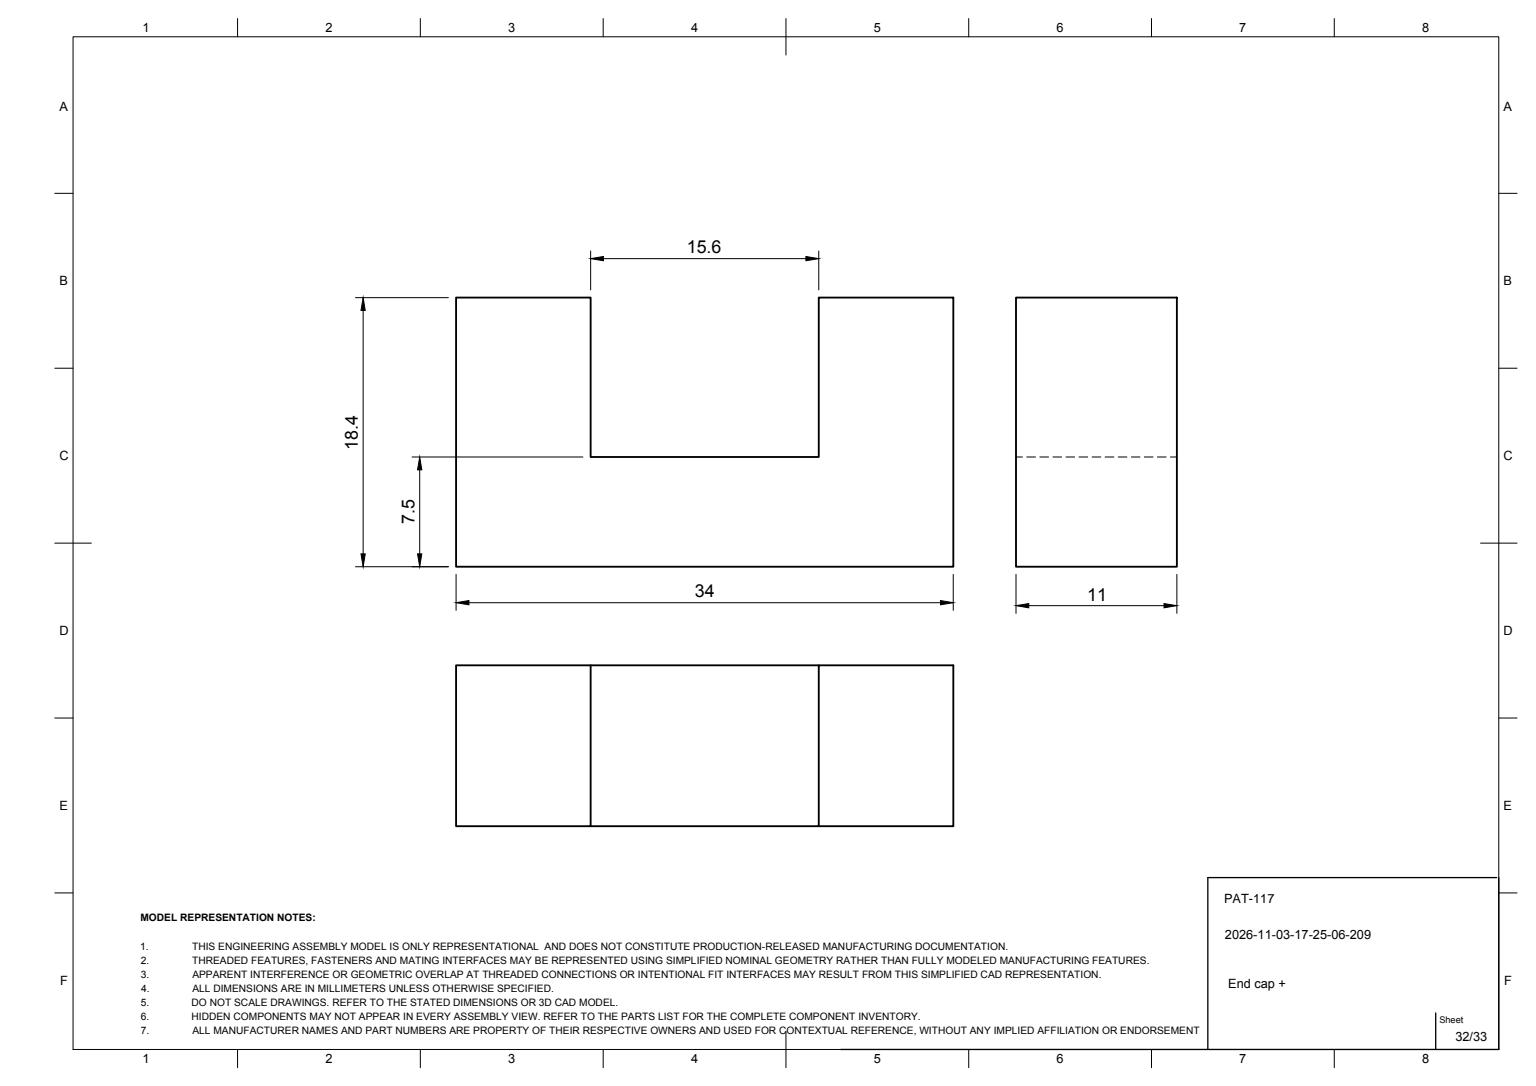
ISO-10303-21;
HEADER;
/* Generated by software containing ST-Developer
 * from STEP Tools, Inc. (www.steptools.com) 
 */

FILE_DESCRIPTION(
/* description */ ('Counterbalanced vertical column'),
/* implementation_level */ '2;1');

FILE_NAME(
/* name */ 'End cap +.step',
/* time_stamp */ '2026-10-29T16:47:22-07:00',
/* author */ (''),
/* organization */ (''),
/* preprocessor_version */ 'ST-DEVELOPER v20.2',
/* originating_system */ 'Autodesk Translation Framework v15.17.0.0',
/* authorisation */ '');

FILE_SCHEMA (('AUTOMOTIVE_DESIGN { 1 0 10303 214 3 1 1 }'));
ENDSEC;

DATA;
#10=MECHANICAL_DESIGN_GEOMETRIC_PRESENTATION_REPRESENTATION('',(#381),#15040);
#311=SHAPE_REPRESENTATION_RELATIONSHIP('SRR','None',#15217,#346);
#346=ADVANCED_BREP_SHAPE_REPRESENTATION('',(#414),#15036);
#381=STYLED_ITEM('',(#15450),#414);
#414=MANIFOLD_SOLID_BREP('Body1',#7106);
#784=PLANE('',#8091);
#785=PLANE('',#8092);
#786=PLANE('',#8093);
#787=PLANE('',#8094);
#788=PLANE('',#8095);
#789=PLANE('',#8096);
#790=PLANE('',#8097);
#791=PLANE('',#8098);
#792=PLANE('',#8099);
#793=PLANE('',#8100);
#1178=FACE_OUTER_BOUND('',#1696,.T.);
#1179=FACE_OUTER_BOUND('',#1697,.T.);
#1180=FACE_OUTER_BOUND('',#1698,.T.);
#1181=FACE_OUTER_BOUND('',#1699,.T.);
#1182=FACE_OUTER_BOUND('',#1700,.T.);
#1183=FACE_OUTER_BOUND('',#1701,.T.);
#1184=FACE_OUTER_BOUND('',#1702,.T.);
#1185=FACE_OUTER_BOUND('',#1703,.T.);
#1186=FACE_OUTER_BOUND('',#1704,.T.);
#1187=FACE_OUTER_BOUND('',#1705,.T.);
#1696=EDGE_LOOP('',(#6354,#6355,#6356,#6357));
#1697=EDGE_LOOP('',(#6358,#6359,#6360,#6361));
#1698=EDGE_LOOP('',(#6362,#6363,#6364,#6365));
#1699=EDGE_LOOP('',(#6366,#6367,#6368,#6369));
#1700=EDGE_LOOP('',(#6370,#6371,#6372,#6373));
#1701=EDGE_LOOP('',(#6374,#6375,#6376,#6377));
#1702=EDGE_LOOP('',(#6378,#6379,#6380,#6381));
#1703=EDGE_LOOP('',(#6382,#6383,#6384,#6385));
#1704=EDGE_LOOP('',(#6386,#6387,#6388,#6389,#6390,#6391,#6392,#6393));
#1705=EDGE_LOOP('',(#6394,#6395,#6396,#6397,#6398,#6399,#6400,#6401));
#2327=LINE('',#14668,#2998);
#2328=LINE('',#14670,#2999);
#2329=LINE('',#14672,#3000);
#2330=LINE('',#14673,#3001);
#2331=LINE('',#14676,#3002);
#2332=LINE('',#14678,#3003);
#2333=LINE('',#14679,#3004);
#2334=LINE('',#14682,#3005);
#2335=LINE('',#14684,#3006);
#2336=LINE('',#14685,#3007);
#2337=LINE('',#14688,#3008);
#2338=LINE('',#14690,#3009);
#2339=LINE('',#14691,#3010);
#2340=LINE('',#14694,#3011);
#2341=LINE('',#14696,#3012);
#2342=LINE('',#14697,#3013);
#2343=LINE('',#14700,#3014);
#2344=LINE('',#14702,#3015);
#2345=LINE('',#14703,#3016);
#2346=LINE('',#14706,#3017);
#2347=LINE('',#14708,#3018);
#2348=LINE('',#14709,#3019);
#2349=LINE('',#14711,#3020);
#2350=LINE('',#14712,#3021);
#2998=VECTOR('',#9985,1.);
#2999=VECTOR('',#9986,1.);
#3000=VECTOR('',#9987,1.);
#3001=VECTOR('',#9988,1.);
#3002=VECTOR('',#9991,1.);
#3003=VECTOR('',#9992,1.);
#3004=VECTOR('',#9993,1.);
#3005=VECTOR('',#9996,1.);
#3006=VECTOR('',#9997,1.);
#3007=VECTOR('',#9998,1.);
#3008=VECTOR('',#10001,1.);
#3009=VECTOR('',#10002,1.);
#3010=VECTOR('',#10003,1.);
#3011=VECTOR('',#10006,1.);
#3012=VECTOR('',#10007,1.);
#3013=VECTOR('',#10008,1.);
#3014=VECTOR('',#10011,1.);
#3015=VECTOR('',#10012,1.);
#3016=VECTOR('',#10013,1.);
#3017=VECTOR('',#10016,1.);
#3018=VECTOR('',#10017,1.);
#3019=VECTOR('',#10018,1.);
#3020=VECTOR('',#10021,1.);
#3021=VECTOR('',#10022,1.);
#3824=VERTEX_POINT('',#14666);
#3825=VERTEX_POINT('',#14667);
#3826=VERTEX_POINT('',#14669);
#3827=VERTEX_POINT('',#14671);
#3828=VERTEX_POINT('',#14675);
#3829=VERTEX_POINT('',#14677);
#3830=VERTEX_POINT('',#14681);
#3831=VERTEX_POINT('',#14683);
#3832=VERTEX_POINT('',#14687);
#3833=VERTEX_POINT('',#14689);
#3834=VERTEX_POINT('',#14693);
#3835=VERTEX_POINT('',#14695);
#3836=VERTEX_POINT('',#14699);
#3837=VERTEX_POINT('',#14701);
#3838=VERTEX_POINT('',#14705);
#3839=VERTEX_POINT('',#14707);
#4678=EDGE_CURVE('',#3824,#3825,#2327,.T.);
#4679=EDGE_CURVE('',#3825,#3826,#2328,.T.);
#4680=EDGE_CURVE('',#3827,#3826,#2329,.T.);
#4681=EDGE_CURVE('',#3824,#3827,#2330,.T.);
#4682=EDGE_CURVE('',#3828,#3824,#2331,.T.);
#4683=EDGE_CURVE('',#3829,#3827,#2332,.T.);
#4684=EDGE_CURVE('',#3828,#3829,#2333,.T.);
#4685=EDGE_CURVE('',#3830,#3828,#2334,.T.);
#4686=EDGE_CURVE('',#3831,#3829,#2335,.T.);
#4687=EDGE_CURVE('',#3830,#3831,#2336,.T.);
#4688=EDGE_CURVE('',#3832,#3830,#2337,.T.);
#4689=EDGE_CURVE('',#3833,#3831,#2338,.T.);
#4690=EDGE_CURVE('',#3832,#3833,#2339,.T.);
#4691=EDGE_CURVE('',#3834,#3832,#2340,.T.);
#4692=EDGE_CURVE('',#3835,#3833,#2341,.T.);
#4693=EDGE_CURVE('',#3834,#3835,#2342,.T.);
#4694=EDGE_CURVE('',#3836,#3834,#2343,.T.);
#4695=EDGE_CURVE('',#3837,#3835,#2344,.T.);
#4696=EDGE_CURVE('',#3836,#3837,#2345,.T.);
#4697=EDGE_CURVE('',#3838,#3836,#2346,.T.);
#4698=EDGE_CURVE('',#3839,#3837,#2347,.T.);
#4699=EDGE_CURVE('',#3838,#3839,#2348,.T.);
#4700=EDGE_CURVE('',#3825,#3838,#2349,.T.);
#4701=EDGE_CURVE('',#3826,#3839,#2350,.T.);
#6354=ORIENTED_EDGE('',*,*,#4678,.T.);
#6355=ORIENTED_EDGE('',*,*,#4679,.T.);
#6356=ORIENTED_EDGE('',*,*,#4680,.F.);
#6357=ORIENTED_EDGE('',*,*,#4681,.F.);
#6358=ORIENTED_EDGE('',*,*,#4682,.T.);
#6359=ORIENTED_EDGE('',*,*,#4681,.T.);
#6360=ORIENTED_EDGE('',*,*,#4683,.F.);
#6361=ORIENTED_EDGE('',*,*,#4684,.F.);
#6362=ORIENTED_EDGE('',*,*,#4685,.T.);
#6363=ORIENTED_EDGE('',*,*,#4684,.T.);
#6364=ORIENTED_EDGE('',*,*,#4686,.F.);
#6365=ORIENTED_EDGE('',*,*,#4687,.F.);
#6366=ORIENTED_EDGE('',*,*,#4688,.T.);
#6367=ORIENTED_EDGE('',*,*,#4687,.T.);
#6368=ORIENTED_EDGE('',*,*,#4689,.F.);
#6369=ORIENTED_EDGE('',*,*,#4690,.F.);
#6370=ORIENTED_EDGE('',*,*,#4691,.T.);
#6371=ORIENTED_EDGE('',*,*,#4690,.T.);
#6372=ORIENTED_EDGE('',*,*,#4692,.F.);
#6373=ORIENTED_EDGE('',*,*,#4693,.F.);
#6374=ORIENTED_EDGE('',*,*,#4694,.T.);
#6375=ORIENTED_EDGE('',*,*,#4693,.T.);
#6376=ORIENTED_EDGE('',*,*,#4695,.F.);
#6377=ORIENTED_EDGE('',*,*,#4696,.F.);
#6378=ORIENTED_EDGE('',*,*,#4697,.T.);
#6379=ORIENTED_EDGE('',*,*,#4696,.T.);
#6380=ORIENTED_EDGE('',*,*,#4698,.F.);
#6381=ORIENTED_EDGE('',*,*,#4699,.F.);
#6382=ORIENTED_EDGE('',*,*,#4700,.T.);
#6383=ORIENTED_EDGE('',*,*,#4699,.T.);
#6384=ORIENTED_EDGE('',*,*,#4701,.F.);
#6385=ORIENTED_EDGE('',*,*,#4679,.F.);
#6386=ORIENTED_EDGE('',*,*,#4701,.T.);
#6387=ORIENTED_EDGE('',*,*,#4698,.T.);
#6388=ORIENTED_EDGE('',*,*,#4695,.T.);
#6389=ORIENTED_EDGE('',*,*,#4692,.T.);
#6390=ORIENTED_EDGE('',*,*,#4689,.T.);
#6391=ORIENTED_EDGE('',*,*,#4686,.T.);
#6392=ORIENTED_EDGE('',*,*,#4683,.T.);
#6393=ORIENTED_EDGE('',*,*,#4680,.T.);
#6394=ORIENTED_EDGE('',*,*,#4700,.F.);
#6395=ORIENTED_EDGE('',*,*,#4678,.F.);
#6396=ORIENTED_EDGE('',*,*,#4682,.F.);
#6397=ORIENTED_EDGE('',*,*,#4685,.F.);
#6398=ORIENTED_EDGE('',*,*,#4688,.F.);
#6399=ORIENTED_EDGE('',*,*,#4691,.F.);
#6400=ORIENTED_EDGE('',*,*,#4694,.F.);
#6401=ORIENTED_EDGE('',*,*,#4697,.F.);
#7020=ADVANCED_FACE('',(#1178),#784,.T.);
#7021=ADVANCED_FACE('',(#1179),#785,.T.);
#7022=ADVANCED_FACE('',(#1180),#786,.T.);
#7023=ADVANCED_FACE('',(#1181),#787,.T.);
#7024=ADVANCED_FACE('',(#1182),#788,.T.);
#7025=ADVANCED_FACE('',(#1183),#789,.T.);
#7026=ADVANCED_FACE('',(#1184),#790,.T.);
#7027=ADVANCED_FACE('',(#1185),#791,.T.);
#7028=ADVANCED_FACE('',(#1186),#792,.T.);
#7029=ADVANCED_FACE('',(#1187),#793,.F.);
#7106=CLOSED_SHELL('',(#7020,#7021,#7022,#7023,#7024,#7025,#7026,#7027,
#7028,#7029));
#8090=AXIS2_PLACEMENT_3D('',#14664,#9981,#9982);
#8091=AXIS2_PLACEMENT_3D('',#14665,#9983,#9984);
#8092=AXIS2_PLACEMENT_3D('',#14674,#9989,#9990);
#8093=AXIS2_PLACEMENT_3D('',#14680,#9994,#9995);
#8094=AXIS2_PLACEMENT_3D('',#14686,#9999,#10000);
#8095=AXIS2_PLACEMENT_3D('',#14692,#10004,#10005);
#8096=AXIS2_PLACEMENT_3D('',#14698,#10009,#10010);
#8097=AXIS2_PLACEMENT_3D('',#14704,#10014,#10015);
#8098=AXIS2_PLACEMENT_3D('',#14710,#10019,#10020);
#8099=AXIS2_PLACEMENT_3D('',#14713,#10023,#10024);
#8100=AXIS2_PLACEMENT_3D('',#14714,#10025,#10026);
#9981=DIRECTION('axis',(0.,0.,1.));
#9982=DIRECTION('refdir',(1.,0.,0.));
#9983=DIRECTION('center_axis',(0.,0.,1.));
#9984=DIRECTION('ref_axis',(0.,-1.,0.));
#9985=DIRECTION('',(0.,-1.,0.));
#9986=DIRECTION('',(1.,0.,0.));
#9987=DIRECTION('',(0.,-1.,0.));
#9988=DIRECTION('',(1.,0.,0.));
#9989=DIRECTION('center_axis',(0.,1.,0.));
#9990=DIRECTION('ref_axis',(0.,0.,1.));
#9991=DIRECTION('',(0.,0.,1.));
#9992=DIRECTION('',(0.,0.,1.));
#9993=DIRECTION('',(1.,0.,0.));
#9994=DIRECTION('center_axis',(0.,0.,-1.));
#9995=DIRECTION('ref_axis',(0.,1.,0.));
#9996=DIRECTION('',(0.,1.,0.));
#9997=DIRECTION('',(0.,1.,0.));
#9998=DIRECTION('',(1.,0.,0.));
#9999=DIRECTION('center_axis',(0.,-1.,0.));
#10000=DIRECTION('ref_axis',(0.,0.,-1.));
#10001=DIRECTION('',(0.,0.,-1.));
#10002=DIRECTION('',(0.,0.,-1.));
#10003=DIRECTION('',(1.,0.,0.));
#10004=DIRECTION('center_axis',(0.,0.,-1.));
#10005=DIRECTION('ref_axis',(0.,1.,0.));
#10006=DIRECTION('',(0.,1.,0.));
#10007=DIRECTION('',(0.,1.,0.));
#10008=DIRECTION('',(1.,0.,0.));
#10009=DIRECTION('center_axis',(0.,1.,0.));
#10010=DIRECTION('ref_axis',(0.,0.,1.));
#10011=DIRECTION('',(0.,0.,1.));
#10012=DIRECTION('',(0.,0.,1.));
#10013=DIRECTION('',(1.,0.,0.));
#10014=DIRECTION('center_axis',(0.,0.,-1.));
#10015=DIRECTION('ref_axis',(0.,1.,0.));
#10016=DIRECTION('',(0.,1.,0.));
#10017=DIRECTION('',(0.,1.,0.));
#10018=DIRECTION('',(1.,0.,0.));
#10019=DIRECTION('center_axis',(0.,-1.,0.));
#10020=DIRECTION('ref_axis',(0.,0.,-1.));
#10021=DIRECTION('',(0.,0.,-1.));
#10022=DIRECTION('',(0.,0.,-1.));
#10023=DIRECTION('center_axis',(1.,0.,0.));
#10024=DIRECTION('ref_axis',(0.,0.,-1.));
#10025=DIRECTION('center_axis',(1.,0.,0.));
#10026=DIRECTION('ref_axis',(0.,0.,-1.));
#14664=CARTESIAN_POINT('',(0.,0.,0.));
#14665=CARTESIAN_POINT('Origin',(1.97,1.7,2.3));
#14666=CARTESIAN_POINT('',(1.97,1.7,2.3));
#14667=CARTESIAN_POINT('',(1.97,-1.7,2.3));
#14668=CARTESIAN_POINT('',(1.97,1.7,2.3));
#14669=CARTESIAN_POINT('',(3.07,-1.7,2.3));
#14670=CARTESIAN_POINT('',(1.97,-1.7,2.3));
#14671=CARTESIAN_POINT('',(3.07,1.7,2.3));
#14672=CARTESIAN_POINT('',(3.07,1.7,2.3));
#14673=CARTESIAN_POINT('',(1.97,1.7,2.3));
#14674=CARTESIAN_POINT('Origin',(1.97,1.7,0.46));
#14675=CARTESIAN_POINT('',(1.97,1.7,0.46));
#14676=CARTESIAN_POINT('',(1.97,1.7,0.46));
#14677=CARTESIAN_POINT('',(3.07,1.7,0.46));
#14678=CARTESIAN_POINT('',(3.07,1.7,0.46));
#14679=CARTESIAN_POINT('',(1.97,1.7,0.46));
#14680=CARTESIAN_POINT('Origin',(1.97,0.78,0.46));
#14681=CARTESIAN_POINT('',(1.97,0.78,0.46));
#14682=CARTESIAN_POINT('',(1.97,0.78,0.46));
#14683=CARTESIAN_POINT('',(3.07,0.78,0.46));
#14684=CARTESIAN_POINT('',(3.07,0.78,0.46));
#14685=CARTESIAN_POINT('',(1.97,0.78,0.46));
#14686=CARTESIAN_POINT('Origin',(1.97,0.78,1.55));
#14687=CARTESIAN_POINT('',(1.97,0.78,1.55));
#14688=CARTESIAN_POINT('',(1.97,0.78,1.55));
#14689=CARTESIAN_POINT('',(3.07,0.78,1.55));
#14690=CARTESIAN_POINT('',(3.07,0.78,1.55));
#14691=CARTESIAN_POINT('',(1.97,0.78,1.55));
#14692=CARTESIAN_POINT('Origin',(1.97,-0.78,1.55));
#14693=CARTESIAN_POINT('',(1.97,-0.78,1.55));
#14694=CARTESIAN_POINT('',(1.97,-0.78,1.55));
#14695=CARTESIAN_POINT('',(3.07,-0.78,1.55));
#14696=CARTESIAN_POINT('',(3.07,-0.78,1.55));
#14697=CARTESIAN_POINT('',(1.97,-0.78,1.55));
#14698=CARTESIAN_POINT('Origin',(1.97,-0.78,0.46));
#14699=CARTESIAN_POINT('',(1.97,-0.78,0.46));
#14700=CARTESIAN_POINT('',(1.97,-0.78,0.46));
#14701=CARTESIAN_POINT('',(3.07,-0.78,0.46));
#14702=CARTESIAN_POINT('',(3.07,-0.78,0.46));
#14703=CARTESIAN_POINT('',(1.97,-0.78,0.46));
#14704=CARTESIAN_POINT('Origin',(1.97,-1.7,0.46));
#14705=CARTESIAN_POINT('',(1.97,-1.7,0.46));
#14706=CARTESIAN_POINT('',(1.97,-1.7,0.46));
#14707=CARTESIAN_POINT('',(3.07,-1.7,0.46));
#14708=CARTESIAN_POINT('',(3.07,-1.7,0.46));
#14709=CARTESIAN_POINT('',(1.97,-1.7,0.46));
#14710=CARTESIAN_POINT('Origin',(1.97,-1.7,2.3));
#14711=CARTESIAN_POINT('',(1.97,-1.7,2.3));
#14712=CARTESIAN_POINT('',(3.07,-1.7,2.3));
#14713=CARTESIAN_POINT('Origin',(3.07,0.,1.38));
#14714=CARTESIAN_POINT('Origin',(1.97,0.,1.38));
#14996=UNCERTAINTY_MEASURE_WITH_UNIT(LENGTH_MEASURE(0.001),#15041,
'DISTANCE_ACCURACY_VALUE',
'Maximum model space distance between geometric entities at asserted c
onnectivities');
#15000=UNCERTAINTY_MEASURE_WITH_UNIT(LENGTH_MEASURE(0.001),#15041,
'DISTANCE_ACCURACY_VALUE',
'Maximum model space distance between geometric entities at asserted c
onnectivities');
#15036=(
GEOMETRIC_REPRESENTATION_CONTEXT(3)
GLOBAL_UNCERTAINTY_ASSIGNED_CONTEXT((#14996))
GLOBAL_UNIT_ASSIGNED_CONTEXT((#15041,#15043,#15044))
REPRESENTATION_CONTEXT('','3D')
);
#15040=(
GEOMETRIC_REPRESENTATION_CONTEXT(3)
GLOBAL_UNCERTAINTY_ASSIGNED_CONTEXT((#15000))
GLOBAL_UNIT_ASSIGNED_CONTEXT((#15041,#15043,#15044))
REPRESENTATION_CONTEXT('','3D')
);
#15041=(
LENGTH_UNIT()
NAMED_UNIT(*)
SI_UNIT(.CENTI.,.METRE.)
);
#15043=(
NAMED_UNIT(*)
PLANE_ANGLE_UNIT()
SI_UNIT($,.RADIAN.)
);
#15044=(
NAMED_UNIT(*)
SI_UNIT($,.STERADIAN.)
SOLID_ANGLE_UNIT()
);
#15080=SHAPE_DEFINITION_REPRESENTATION(#15119,#15217);
#15119=PRODUCT_DEFINITION_SHAPE('',$,#15257);
#15217=SHAPE_REPRESENTATION('',(#8090),#15036);
#15221=PRODUCT_DEFINITION_CONTEXT('part definition',#15340,'design');
#15257=PRODUCT_DEFINITION('End cap +','End cap +',#15296,#15221);
#15296=PRODUCT_DEFINITION_FORMATION('',$,#15377);
#15340=APPLICATION_CONTEXT(
'Core Data for Automotive Mechanical Design Process');
#15341=PRODUCT_CONTEXT('part definition',#15340,'mechanical');
#15377=PRODUCT('End cap +','End cap +','End cap +',(#15341));
#15444=COLOUR_RGB('Sky Blue',0.24,0.69,0.87);
#15445=FILL_AREA_STYLE_COLOUR('',#15444);
#15446=FILL_AREA_STYLE('',(#15445));
#15447=SURFACE_STYLE_FILL_AREA(#15446);
#15448=SURFACE_SIDE_STYLE('',(#15447));
#15449=SURFACE_STYLE_USAGE(.BOTH.,#15448);
#15450=PRESENTATION_STYLE_ASSIGNMENT((#15449));
ENDSEC;
END-ISO-10303-21;
